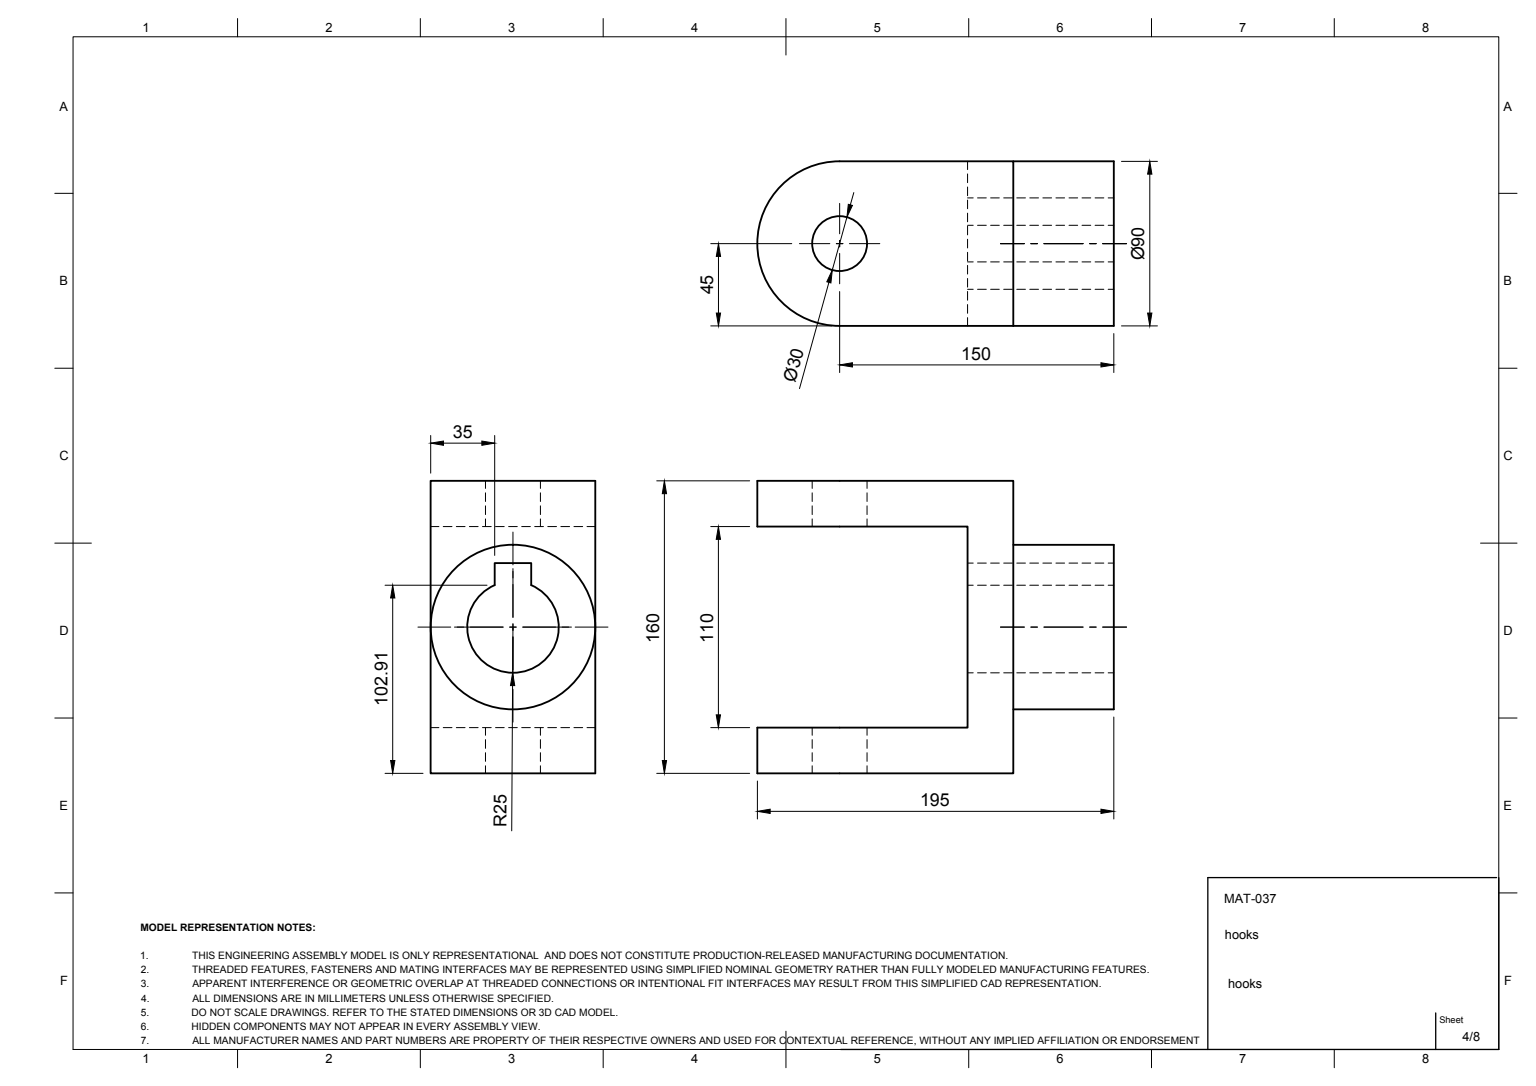
ISO-10303-21;
HEADER;
/* Generated by software containing ST-Developer
 * from STEP Tools, Inc. (www.steptools.com) 
 */

FILE_DESCRIPTION(
/* description */ ('STEP AP214'),
/* implementation_level */ '2;1');

FILE_NAME(
/* name */ 'hooks.step',
/* time_stamp */ '2026-11-14T21:09:07-08:00',
/* author */ (''),
/* organization */ (''),
/* preprocessor_version */ 'ST-DEVELOPER v20.2',
/* originating_system */ 'Autodesk Translation Framework v15.17.0.0',
/* authorisation */ '');

FILE_SCHEMA (('AUTOMOTIVE_DESIGN { 1 0 10303 214 3 1 1 }'));
ENDSEC;

DATA;
#10=MECHANICAL_DESIGN_GEOMETRIC_PRESENTATION_REPRESENTATION('',(#79),#2059);
#65=SHAPE_REPRESENTATION_RELATIONSHIP('SRR','None',#2095,#72);
#72=ADVANCED_BREP_SHAPE_REPRESENTATION('',(#86),#2053);
#79=STYLED_ITEM('',(#2139),#86);
#86=MANIFOLD_SOLID_BREP('Body1',#976);
#96=PLANE('',#1092);
#97=PLANE('',#1093);
#98=PLANE('',#1094);
#99=PLANE('',#1095);
#100=PLANE('',#1097);
#101=PLANE('',#1098);
#102=PLANE('',#1100);
#103=PLANE('',#1102);
#104=PLANE('',#1103);
#105=PLANE('',#1105);
#106=PLANE('',#1108);
#107=PLANE('',#1109);
#108=PLANE('',#1110);
#131=FACE_BOUND('',#234,.T.);
#132=FACE_BOUND('',#237,.T.);
#133=FACE_BOUND('',#239,.T.);
#134=FACE_BOUND('',#241,.T.);
#135=FACE_BOUND('',#243,.T.);
#136=FACE_BOUND('',#245,.T.);
#164=FACE_OUTER_BOUND('',#226,.T.);
#165=FACE_OUTER_BOUND('',#227,.T.);
#166=FACE_OUTER_BOUND('',#228,.T.);
#167=FACE_OUTER_BOUND('',#229,.T.);
#168=FACE_OUTER_BOUND('',#230,.T.);
#169=FACE_OUTER_BOUND('',#231,.T.);
#170=FACE_OUTER_BOUND('',#232,.T.);
#171=FACE_OUTER_BOUND('',#233,.T.);
#172=FACE_OUTER_BOUND('',#235,.T.);
#173=FACE_OUTER_BOUND('',#236,.T.);
#174=FACE_OUTER_BOUND('',#238,.T.);
#175=FACE_OUTER_BOUND('',#240,.T.);
#176=FACE_OUTER_BOUND('',#242,.T.);
#177=FACE_OUTER_BOUND('',#244,.T.);
#178=FACE_OUTER_BOUND('',#246,.T.);
#179=FACE_OUTER_BOUND('',#247,.T.);
#180=FACE_OUTER_BOUND('',#248,.T.);
#181=FACE_OUTER_BOUND('',#249,.T.);
#182=FACE_OUTER_BOUND('',#250,.T.);
#226=EDGE_LOOP('',(#685,#686,#687,#688));
#227=EDGE_LOOP('',(#689,#690,#691,#692));
#228=EDGE_LOOP('',(#693,#694,#695,#696));
#229=EDGE_LOOP('',(#697,#698,#699,#700,#701));
#230=EDGE_LOOP('',(#702,#703,#704,#705,#706,#707,#708,#709,#710));
#231=EDGE_LOOP('',(#711,#712,#713,#714,#715,#716,#717,#718,#719));
#232=EDGE_LOOP('',(#720,#721,#722,#723));
#233=EDGE_LOOP('',(#724,#725,#726,#727));
#234=EDGE_LOOP('',(#728));
#235=EDGE_LOOP('',(#729,#730,#731,#732));
#236=EDGE_LOOP('',(#733,#734,#735,#736));
#237=EDGE_LOOP('',(#737));
#238=EDGE_LOOP('',(#738,#739,#740,#741));
#239=EDGE_LOOP('',(#742));
#240=EDGE_LOOP('',(#743,#744,#745,#746));
#241=EDGE_LOOP('',(#747,#748,#749,#750));
#242=EDGE_LOOP('',(#751,#752,#753,#754));
#243=EDGE_LOOP('',(#755));
#244=EDGE_LOOP('',(#756));
#245=EDGE_LOOP('',(#757,#758,#759,#760));
#246=EDGE_LOOP('',(#761,#762,#763,#764));
#247=EDGE_LOOP('',(#765,#766,#767,#768));
#248=EDGE_LOOP('',(#769,#770,#771,#772));
#249=EDGE_LOOP('',(#773,#774,#775,#776));
#250=EDGE_LOOP('',(#777,#778,#779,#780));
#292=LINE('',#1587,#357);
#293=LINE('',#1593,#358);
#294=LINE('',#1600,#359);
#295=LINE('',#1603,#360);
#296=LINE('',#1609,#361);
#297=LINE('',#1615,#362);
#298=LINE('',#1617,#363);
#299=LINE('',#1619,#364);
#300=LINE('',#1621,#365);
#301=LINE('',#1623,#366);
#302=LINE('',#1625,#367);
#303=LINE('',#1627,#368);
#304=LINE('',#1628,#369);
#305=LINE('',#1629,#370);
#306=LINE('',#1633,#371);
#307=LINE('',#1635,#372);
#308=LINE('',#1636,#373);
#309=LINE('',#1638,#374);
#310=LINE('',#1640,#375);
#311=LINE('',#1642,#376);
#312=LINE('',#1644,#377);
#313=LINE('',#1646,#378);
#314=LINE('',#1647,#379);
#315=LINE('',#1649,#380);
#316=LINE('',#1653,#381);
#317=LINE('',#1658,#382);
#318=LINE('',#1660,#383);
#319=LINE('',#1662,#384);
#320=LINE('',#1664,#385);
#321=LINE('',#1665,#386);
#322=LINE('',#1670,#387);
#323=LINE('',#1672,#388);
#324=LINE('',#1673,#389);
#325=LINE('',#1677,#390);
#326=LINE('',#1679,#391);
#357=VECTOR('',#1226,15.0000000000001);
#358=VECTOR('',#1233,15.0000000000001);
#359=VECTOR('',#1240,1000.);
#360=VECTOR('',#1243,1000.);
#361=VECTOR('',#1248,45.0000000000003);
#362=VECTOR('',#1255,1000.);
#363=VECTOR('',#1256,1000.);
#364=VECTOR('',#1257,1000.);
#365=VECTOR('',#1258,1000.);
#366=VECTOR('',#1259,1000.);
#367=VECTOR('',#1260,1000.);
#368=VECTOR('',#1261,1000.);
#369=VECTOR('',#1262,1000.);
#370=VECTOR('',#1263,1000.);
#371=VECTOR('',#1266,1000.);
#372=VECTOR('',#1267,1000.);
#373=VECTOR('',#1268,1000.);
#374=VECTOR('',#1269,1000.);
#375=VECTOR('',#1270,1000.);
#376=VECTOR('',#1271,1000.);
#377=VECTOR('',#1272,1000.);
#378=VECTOR('',#1273,1000.);
#379=VECTOR('',#1274,1000.);
#380=VECTOR('',#1277,1000.);
#381=VECTOR('',#1284,1000.);
#382=VECTOR('',#1293,1000.);
#383=VECTOR('',#1296,1000.);
#384=VECTOR('',#1297,1000.);
#385=VECTOR('',#1298,1000.);
#386=VECTOR('',#1299,1000.);
#387=VECTOR('',#1306,1000.);
#388=VECTOR('',#1307,1000.);
#389=VECTOR('',#1308,1000.);
#390=VECTOR('',#1315,1000.);
#391=VECTOR('',#1318,1000.);
#426=CIRCLE('',#1080,15.0000000000001);
#427=CIRCLE('',#1081,15.0000000000001);
#428=CIRCLE('',#1083,15.0000000000001);
#429=CIRCLE('',#1084,15.0000000000001);
#430=CIRCLE('',#1086,25.0000000000002);
#431=CIRCLE('',#1087,25.0000000000002);
#432=CIRCLE('',#1089,45.0000000000003);
#433=CIRCLE('',#1090,45.0000000000003);
#434=CIRCLE('',#1091,45.0000000000003);
#435=CIRCLE('',#1096,45.0000000000003);
#436=CIRCLE('',#1099,45.0000000000003);
#437=CIRCLE('',#1101,45.0000000000003);
#438=CIRCLE('',#1104,45.0000000000003);
#470=VERTEX_POINT('',#1584);
#471=VERTEX_POINT('',#1586);
#472=VERTEX_POINT('',#1590);
#473=VERTEX_POINT('',#1592);
#474=VERTEX_POINT('',#1596);
#475=VERTEX_POINT('',#1597);
#476=VERTEX_POINT('',#1599);
#477=VERTEX_POINT('',#1601);
#478=VERTEX_POINT('',#1605);
#479=VERTEX_POINT('',#1606);
#480=VERTEX_POINT('',#1608);
#481=VERTEX_POINT('',#1613);
#482=VERTEX_POINT('',#1614);
#483=VERTEX_POINT('',#1616);
#484=VERTEX_POINT('',#1618);
#485=VERTEX_POINT('',#1620);
#486=VERTEX_POINT('',#1622);
#487=VERTEX_POINT('',#1624);
#488=VERTEX_POINT('',#1626);
#489=VERTEX_POINT('',#1631);
#490=VERTEX_POINT('',#1632);
#491=VERTEX_POINT('',#1634);
#492=VERTEX_POINT('',#1637);
#493=VERTEX_POINT('',#1639);
#494=VERTEX_POINT('',#1641);
#495=VERTEX_POINT('',#1643);
#496=VERTEX_POINT('',#1645);
#497=VERTEX_POINT('',#1661);
#498=VERTEX_POINT('',#1663);
#499=VERTEX_POINT('',#1669);
#500=VERTEX_POINT('',#1671);
#553=EDGE_CURVE('',#470,#470,#426,.T.);
#554=EDGE_CURVE('',#470,#471,#292,.T.);
#555=EDGE_CURVE('',#471,#471,#427,.T.);
#556=EDGE_CURVE('',#472,#472,#428,.T.);
#557=EDGE_CURVE('',#472,#473,#293,.T.);
#558=EDGE_CURVE('',#473,#473,#429,.T.);
#559=EDGE_CURVE('',#474,#475,#430,.T.);
#560=EDGE_CURVE('',#476,#474,#294,.T.);
#561=EDGE_CURVE('',#476,#477,#431,.T.);
#562=EDGE_CURVE('',#475,#477,#295,.T.);
#563=EDGE_CURVE('',#478,#479,#432,.T.);
#564=EDGE_CURVE('',#478,#480,#296,.T.);
#565=EDGE_CURVE('',#480,#480,#433,.T.);
#566=EDGE_CURVE('',#479,#478,#434,.T.);
#567=EDGE_CURVE('',#481,#482,#297,.T.);
#568=EDGE_CURVE('',#482,#483,#298,.T.);
#569=EDGE_CURVE('',#483,#484,#299,.T.);
#570=EDGE_CURVE('',#485,#484,#300,.T.);
#571=EDGE_CURVE('',#485,#486,#301,.T.);
#572=EDGE_CURVE('',#486,#487,#302,.T.);
#573=EDGE_CURVE('',#487,#488,#303,.T.);
#574=EDGE_CURVE('',#488,#478,#304,.T.);
#575=EDGE_CURVE('',#478,#481,#305,.T.);
#576=EDGE_CURVE('',#489,#490,#306,.T.);
#577=EDGE_CURVE('',#491,#489,#307,.T.);
#578=EDGE_CURVE('',#479,#491,#308,.T.);
#579=EDGE_CURVE('',#492,#479,#309,.T.);
#580=EDGE_CURVE('',#493,#492,#310,.T.);
#581=EDGE_CURVE('',#494,#493,#311,.T.);
#582=EDGE_CURVE('',#495,#494,#312,.T.);
#583=EDGE_CURVE('',#495,#496,#313,.T.);
#584=EDGE_CURVE('',#490,#496,#314,.T.);
#585=EDGE_CURVE('',#488,#492,#315,.T.);
#586=EDGE_CURVE('',#493,#487,#435,.T.);
#587=EDGE_CURVE('',#481,#491,#316,.T.);
#588=EDGE_CURVE('',#489,#482,#436,.T.);
#589=EDGE_CURVE('',#483,#490,#437,.T.);
#590=EDGE_CURVE('',#484,#496,#317,.T.);
#591=EDGE_CURVE('',#485,#495,#318,.T.);
#592=EDGE_CURVE('',#477,#497,#319,.T.);
#593=EDGE_CURVE('',#498,#476,#320,.T.);
#594=EDGE_CURVE('',#497,#498,#321,.T.);
#595=EDGE_CURVE('',#494,#486,#438,.T.);
#596=EDGE_CURVE('',#499,#475,#322,.T.);
#597=EDGE_CURVE('',#500,#499,#323,.T.);
#598=EDGE_CURVE('',#474,#500,#324,.T.);
#599=EDGE_CURVE('',#497,#499,#325,.T.);
#600=EDGE_CURVE('',#498,#500,#326,.T.);
#685=ORIENTED_EDGE('',*,*,#553,.F.);
#686=ORIENTED_EDGE('',*,*,#554,.T.);
#687=ORIENTED_EDGE('',*,*,#555,.F.);
#688=ORIENTED_EDGE('',*,*,#554,.F.);
#689=ORIENTED_EDGE('',*,*,#556,.F.);
#690=ORIENTED_EDGE('',*,*,#557,.T.);
#691=ORIENTED_EDGE('',*,*,#558,.T.);
#692=ORIENTED_EDGE('',*,*,#557,.F.);
#693=ORIENTED_EDGE('',*,*,#559,.F.);
#694=ORIENTED_EDGE('',*,*,#560,.F.);
#695=ORIENTED_EDGE('',*,*,#561,.T.);
#696=ORIENTED_EDGE('',*,*,#562,.F.);
#697=ORIENTED_EDGE('',*,*,#563,.F.);
#698=ORIENTED_EDGE('',*,*,#564,.T.);
#699=ORIENTED_EDGE('',*,*,#565,.T.);
#700=ORIENTED_EDGE('',*,*,#564,.F.);
#701=ORIENTED_EDGE('',*,*,#566,.F.);
#702=ORIENTED_EDGE('',*,*,#567,.T.);
#703=ORIENTED_EDGE('',*,*,#568,.T.);
#704=ORIENTED_EDGE('',*,*,#569,.T.);
#705=ORIENTED_EDGE('',*,*,#570,.F.);
#706=ORIENTED_EDGE('',*,*,#571,.T.);
#707=ORIENTED_EDGE('',*,*,#572,.T.);
#708=ORIENTED_EDGE('',*,*,#573,.T.);
#709=ORIENTED_EDGE('',*,*,#574,.T.);
#710=ORIENTED_EDGE('',*,*,#575,.T.);
#711=ORIENTED_EDGE('',*,*,#576,.F.);
#712=ORIENTED_EDGE('',*,*,#577,.F.);
#713=ORIENTED_EDGE('',*,*,#578,.F.);
#714=ORIENTED_EDGE('',*,*,#579,.F.);
#715=ORIENTED_EDGE('',*,*,#580,.F.);
#716=ORIENTED_EDGE('',*,*,#581,.F.);
#717=ORIENTED_EDGE('',*,*,#582,.F.);
#718=ORIENTED_EDGE('',*,*,#583,.T.);
#719=ORIENTED_EDGE('',*,*,#584,.F.);
#720=ORIENTED_EDGE('',*,*,#579,.T.);
#721=ORIENTED_EDGE('',*,*,#566,.T.);
#722=ORIENTED_EDGE('',*,*,#574,.F.);
#723=ORIENTED_EDGE('',*,*,#585,.T.);
#724=ORIENTED_EDGE('',*,*,#573,.F.);
#725=ORIENTED_EDGE('',*,*,#586,.F.);
#726=ORIENTED_EDGE('',*,*,#580,.T.);
#727=ORIENTED_EDGE('',*,*,#585,.F.);
#728=ORIENTED_EDGE('',*,*,#558,.F.);
#729=ORIENTED_EDGE('',*,*,#575,.F.);
#730=ORIENTED_EDGE('',*,*,#563,.T.);
#731=ORIENTED_EDGE('',*,*,#578,.T.);
#732=ORIENTED_EDGE('',*,*,#587,.F.);
#733=ORIENTED_EDGE('',*,*,#577,.T.);
#734=ORIENTED_EDGE('',*,*,#588,.T.);
#735=ORIENTED_EDGE('',*,*,#567,.F.);
#736=ORIENTED_EDGE('',*,*,#587,.T.);
#737=ORIENTED_EDGE('',*,*,#553,.T.);
#738=ORIENTED_EDGE('',*,*,#569,.F.);
#739=ORIENTED_EDGE('',*,*,#589,.T.);
#740=ORIENTED_EDGE('',*,*,#584,.T.);
#741=ORIENTED_EDGE('',*,*,#590,.F.);
#742=ORIENTED_EDGE('',*,*,#555,.T.);
#743=ORIENTED_EDGE('',*,*,#583,.F.);
#744=ORIENTED_EDGE('',*,*,#591,.F.);
#745=ORIENTED_EDGE('',*,*,#570,.T.);
#746=ORIENTED_EDGE('',*,*,#590,.T.);
#747=ORIENTED_EDGE('',*,*,#592,.F.);
#748=ORIENTED_EDGE('',*,*,#561,.F.);
#749=ORIENTED_EDGE('',*,*,#593,.F.);
#750=ORIENTED_EDGE('',*,*,#594,.F.);
#751=ORIENTED_EDGE('',*,*,#582,.T.);
#752=ORIENTED_EDGE('',*,*,#595,.T.);
#753=ORIENTED_EDGE('',*,*,#571,.F.);
#754=ORIENTED_EDGE('',*,*,#591,.T.);
#755=ORIENTED_EDGE('',*,*,#556,.T.);
#756=ORIENTED_EDGE('',*,*,#565,.F.);
#757=ORIENTED_EDGE('',*,*,#596,.F.);
#758=ORIENTED_EDGE('',*,*,#597,.F.);
#759=ORIENTED_EDGE('',*,*,#598,.F.);
#760=ORIENTED_EDGE('',*,*,#559,.T.);
#761=ORIENTED_EDGE('',*,*,#586,.T.);
#762=ORIENTED_EDGE('',*,*,#572,.F.);
#763=ORIENTED_EDGE('',*,*,#595,.F.);
#764=ORIENTED_EDGE('',*,*,#581,.T.);
#765=ORIENTED_EDGE('',*,*,#576,.T.);
#766=ORIENTED_EDGE('',*,*,#589,.F.);
#767=ORIENTED_EDGE('',*,*,#568,.F.);
#768=ORIENTED_EDGE('',*,*,#588,.F.);
#769=ORIENTED_EDGE('',*,*,#592,.T.);
#770=ORIENTED_EDGE('',*,*,#599,.T.);
#771=ORIENTED_EDGE('',*,*,#596,.T.);
#772=ORIENTED_EDGE('',*,*,#562,.T.);
#773=ORIENTED_EDGE('',*,*,#594,.T.);
#774=ORIENTED_EDGE('',*,*,#600,.T.);
#775=ORIENTED_EDGE('',*,*,#597,.T.);
#776=ORIENTED_EDGE('',*,*,#599,.F.);
#777=ORIENTED_EDGE('',*,*,#593,.T.);
#778=ORIENTED_EDGE('',*,*,#560,.T.);
#779=ORIENTED_EDGE('',*,*,#598,.T.);
#780=ORIENTED_EDGE('',*,*,#600,.F.);
#901=CYLINDRICAL_SURFACE('',#1079,15.0000000000001);
#902=CYLINDRICAL_SURFACE('',#1082,15.0000000000001);
#903=CYLINDRICAL_SURFACE('',#1085,25.0000000000002);
#904=CYLINDRICAL_SURFACE('',#1088,45.0000000000003);
#905=CYLINDRICAL_SURFACE('',#1106,45.0000000000003);
#906=CYLINDRICAL_SURFACE('',#1107,45.0000000000003);
#927=ADVANCED_FACE('',(#164),#901,.F.);
#928=ADVANCED_FACE('',(#165),#902,.F.);
#929=ADVANCED_FACE('',(#166),#903,.F.);
#930=ADVANCED_FACE('',(#167),#904,.T.);
#931=ADVANCED_FACE('',(#168),#96,.T.);
#932=ADVANCED_FACE('',(#169),#97,.F.);
#933=ADVANCED_FACE('',(#170),#98,.F.);
#934=ADVANCED_FACE('',(#171,#131),#99,.F.);
#935=ADVANCED_FACE('',(#172),#100,.F.);
#936=ADVANCED_FACE('',(#173,#132),#101,.F.);
#937=ADVANCED_FACE('',(#174,#133),#102,.F.);
#938=ADVANCED_FACE('',(#175,#134),#103,.T.);
#939=ADVANCED_FACE('',(#176,#135),#104,.F.);
#940=ADVANCED_FACE('',(#177,#136),#105,.T.);
#941=ADVANCED_FACE('',(#178),#905,.T.);
#942=ADVANCED_FACE('',(#179),#906,.T.);
#943=ADVANCED_FACE('',(#180),#106,.F.);
#944=ADVANCED_FACE('',(#181),#107,.F.);
#945=ADVANCED_FACE('',(#182),#108,.F.);
#976=CLOSED_SHELL('',(#927,#928,#929,#930,#931,#932,#933,#934,#935,#936,
#937,#938,#939,#940,#941,#942,#943,#944,#945));
#1078=AXIS2_PLACEMENT_3D('',#1582,#1220,#1221);
#1079=AXIS2_PLACEMENT_3D('',#1583,#1222,#1223);
#1080=AXIS2_PLACEMENT_3D('',#1585,#1224,#1225);
#1081=AXIS2_PLACEMENT_3D('',#1588,#1227,#1228);
#1082=AXIS2_PLACEMENT_3D('',#1589,#1229,#1230);
#1083=AXIS2_PLACEMENT_3D('',#1591,#1231,#1232);
#1084=AXIS2_PLACEMENT_3D('',#1594,#1234,#1235);
#1085=AXIS2_PLACEMENT_3D('',#1595,#1236,#1237);
#1086=AXIS2_PLACEMENT_3D('',#1598,#1238,#1239);
#1087=AXIS2_PLACEMENT_3D('',#1602,#1241,#1242);
#1088=AXIS2_PLACEMENT_3D('',#1604,#1244,#1245);
#1089=AXIS2_PLACEMENT_3D('',#1607,#1246,#1247);
#1090=AXIS2_PLACEMENT_3D('',#1610,#1249,#1250);
#1091=AXIS2_PLACEMENT_3D('',#1611,#1251,#1252);
#1092=AXIS2_PLACEMENT_3D('',#1612,#1253,#1254);
#1093=AXIS2_PLACEMENT_3D('',#1630,#1264,#1265);
#1094=AXIS2_PLACEMENT_3D('',#1648,#1275,#1276);
#1095=AXIS2_PLACEMENT_3D('',#1650,#1278,#1279);
#1096=AXIS2_PLACEMENT_3D('',#1651,#1280,#1281);
#1097=AXIS2_PLACEMENT_3D('',#1652,#1282,#1283);
#1098=AXIS2_PLACEMENT_3D('',#1654,#1285,#1286);
#1099=AXIS2_PLACEMENT_3D('',#1655,#1287,#1288);
#1100=AXIS2_PLACEMENT_3D('',#1656,#1289,#1290);
#1101=AXIS2_PLACEMENT_3D('',#1657,#1291,#1292);
#1102=AXIS2_PLACEMENT_3D('',#1659,#1294,#1295);
#1103=AXIS2_PLACEMENT_3D('',#1666,#1300,#1301);
#1104=AXIS2_PLACEMENT_3D('',#1667,#1302,#1303);
#1105=AXIS2_PLACEMENT_3D('',#1668,#1304,#1305);
#1106=AXIS2_PLACEMENT_3D('',#1674,#1309,#1310);
#1107=AXIS2_PLACEMENT_3D('',#1675,#1311,#1312);
#1108=AXIS2_PLACEMENT_3D('',#1676,#1313,#1314);
#1109=AXIS2_PLACEMENT_3D('',#1678,#1316,#1317);
#1110=AXIS2_PLACEMENT_3D('',#1680,#1319,#1320);
#1220=DIRECTION('axis',(0.,0.,1.));
#1221=DIRECTION('refdir',(1.,0.,0.));
#1222=DIRECTION('center_axis',(-8.09275762631517E-30,1.,-3.72243739651165E-30));
#1223=DIRECTION('ref_axis',(-3.01247836291004E-59,3.72243739651165E-30,
1.));
#1224=DIRECTION('center_axis',(-8.09237244032629E-30,1.,-3.72243739651165E-30));
#1225=DIRECTION('ref_axis',(-3.01233497983708E-59,3.72243739651165E-30,
1.));
#1226=DIRECTION('',(-8.09275762631517E-30,1.,-3.72243739651165E-30));
#1227=DIRECTION('center_axis',(8.09237244032629E-30,-1.,3.72243739651165E-30));
#1228=DIRECTION('ref_axis',(3.01233497983708E-59,-3.72243739651165E-30,
-1.));
#1229=DIRECTION('center_axis',(-8.09275762631517E-30,1.,-3.72243739651165E-30));
#1230=DIRECTION('ref_axis',(-3.01247836291004E-59,3.72243739651165E-30,
1.));
#1231=DIRECTION('center_axis',(-8.09237244032629E-30,1.,-3.72243739651165E-30));
#1232=DIRECTION('ref_axis',(-3.01233497983708E-59,3.72243739651165E-30,
1.));
#1233=DIRECTION('',(-8.09275762631517E-30,1.,-3.72243739651165E-30));
#1234=DIRECTION('center_axis',(-8.09275762631517E-30,1.,-3.72243739651165E-30));
#1235=DIRECTION('ref_axis',(-3.01247836291004E-59,3.72243739651165E-30,
1.));
#1236=DIRECTION('center_axis',(1.,-7.90786835165394E-30,1.38777878078144E-17));
#1237=DIRECTION('ref_axis',(-7.96009957174572E-30,-1.,3.7364106986726E-15));
#1238=DIRECTION('center_axis',(1.,-7.90786835165394E-30,1.38777878078144E-17));
#1239=DIRECTION('ref_axis',(1.38777878078144E-17,-1.09743718996384E-46,
-1.));
#1240=DIRECTION('',(-1.,7.90786835165394E-30,-1.38777878078144E-17));
#1241=DIRECTION('center_axis',(1.,-8.05423902742737E-30,1.04083408558608E-17));
#1242=DIRECTION('ref_axis',(1.04083408558608E-17,-8.38312651320406E-47,
-1.));
#1243=DIRECTION('',(1.,-7.90786835165394E-30,1.38777878078144E-17));
#1244=DIRECTION('center_axis',(1.,-7.90786835165394E-30,1.38777878078144E-17));
#1245=DIRECTION('ref_axis',(1.38777878078144E-17,-1.09743718996384E-46,
-1.));
#1246=DIRECTION('center_axis',(1.,-7.90786835165394E-30,1.38777878078144E-17));
#1247=DIRECTION('ref_axis',(1.38777878078144E-17,-1.09743718996384E-46,
-1.));
#1248=DIRECTION('',(-1.,7.90786835165394E-30,-1.38777878078144E-17));
#1249=DIRECTION('center_axis',(1.,-7.90786835165394E-30,1.38777878078144E-17));
#1250=DIRECTION('ref_axis',(1.38777878078144E-17,-1.09743718996384E-46,
-1.));
#1251=DIRECTION('center_axis',(1.,-7.90786835165394E-30,1.38777878078144E-17));
#1252=DIRECTION('ref_axis',(1.38777878078144E-17,-1.09743718996384E-46,
-1.));
#1253=DIRECTION('center_axis',(-1.38777878078144E-17,-3.94430452610503E-30,
1.));
#1254=DIRECTION('ref_axis',(1.,-7.90786835165394E-30,1.38777878078144E-17));
#1255=DIRECTION('',(1.,-7.90786835165394E-30,1.38777878078144E-17));
#1256=DIRECTION('',(-8.09275762631517E-30,1.,-3.72243739651165E-30));
#1257=DIRECTION('',(-1.,7.90786835165394E-30,-1.38777878078144E-17));
#1258=DIRECTION('',(8.09275762631517E-30,-1.,3.72243739651165E-30));
#1259=DIRECTION('',(1.,-7.90786835165394E-30,1.38777878078144E-17));
#1260=DIRECTION('',(-8.09275762631517E-30,1.,-3.72243739651165E-30));
#1261=DIRECTION('',(-1.,7.90786835165394E-30,-1.38777878078144E-17));
#1262=DIRECTION('',(8.09275762631517E-30,-1.,3.72243739651165E-30));
#1263=DIRECTION('',(8.09275762631517E-30,-1.,3.72243739651165E-30));
#1264=DIRECTION('center_axis',(-1.38777878078144E-17,-3.94430452610503E-30,
1.));
#1265=DIRECTION('ref_axis',(1.,-7.90786835165394E-30,1.38777878078144E-17));
#1266=DIRECTION('',(-8.09275762631517E-30,1.,-3.72243739651165E-30));
#1267=DIRECTION('',(1.,-8.05423902742737E-30,1.04083408558608E-17));
#1268=DIRECTION('',(8.09275762631517E-30,-1.,3.72243739651165E-30));
#1269=DIRECTION('',(8.09275762631517E-30,-1.,3.72243739651165E-30));
#1270=DIRECTION('',(-1.,7.90786835165394E-30,-1.38777878078144E-17));
#1271=DIRECTION('',(-8.09275762631517E-30,1.,-3.72243739651165E-30));
#1272=DIRECTION('',(1.,-7.90786835165394E-30,1.38777878078144E-17));
#1273=DIRECTION('',(8.09275762631517E-30,-1.,3.72243739651165E-30));
#1274=DIRECTION('',(-1.,7.90786835165394E-30,-1.38777878078144E-17));
#1275=DIRECTION('center_axis',(1.,-8.05423902742737E-30,1.38777878078144E-17));
#1276=DIRECTION('ref_axis',(1.38777878078144E-17,3.94430452610503E-30,-1.));
#1277=DIRECTION('',(1.04083408558608E-17,3.77174120308794E-30,-1.));
#1278=DIRECTION('center_axis',(8.09237244032629E-30,-1.,-3.94430452610503E-30));
#1279=DIRECTION('ref_axis',(1.38777878078144E-17,3.94430452610503E-30,-1.));
#1280=DIRECTION('center_axis',(8.09275762631517E-30,-1.,3.72243739651165E-30));
#1281=DIRECTION('ref_axis',(-9.8532293435482E-14,3.72243739651085E-30,1.));
#1282=DIRECTION('center_axis',(1.,-8.05423902742737E-30,1.38777878078144E-17));
#1283=DIRECTION('ref_axis',(1.38777878078144E-17,3.94430452610503E-30,-1.));
#1284=DIRECTION('',(1.04083408558608E-17,3.77174120308794E-30,-1.));
#1285=DIRECTION('center_axis',(-8.09237244032629E-30,1.,3.94430452610503E-30));
#1286=DIRECTION('ref_axis',(-1.38777878078144E-17,-3.94430452610503E-30,
1.));
#1287=DIRECTION('center_axis',(8.09237244032629E-30,-1.,3.72243739651165E-30));
#1288=DIRECTION('ref_axis',(-1.87350135405494E-13,3.72243739651013E-30,
1.));
#1289=DIRECTION('center_axis',(8.09237244032629E-30,-1.,-3.94430452610503E-30));
#1290=DIRECTION('ref_axis',(1.38777878078144E-17,3.94430452610503E-30,-1.));
#1291=DIRECTION('center_axis',(-8.09237244032629E-30,1.,-3.72243739651165E-30));
#1292=DIRECTION('ref_axis',(-1.19040579862585E-13,-3.72243739651261E-30,
-1.));
#1293=DIRECTION('',(1.04083408558608E-17,3.77174120308794E-30,-1.));
#1294=DIRECTION('center_axis',(1.,-8.05423902742737E-30,1.38777878078144E-17));
#1295=DIRECTION('ref_axis',(1.38777878078144E-17,3.94430452610503E-30,-1.));
#1296=DIRECTION('',(1.04083408558608E-17,3.77174120308794E-30,-1.));
#1297=DIRECTION('',(-8.09275762631517E-30,1.,-3.72243739651165E-30));
#1298=DIRECTION('',(8.09275762631517E-30,-1.,3.72243739651165E-30));
#1299=DIRECTION('',(-1.38777878078144E-17,-3.94430452610503E-30,1.));
#1300=DIRECTION('center_axis',(-8.09237244032629E-30,1.,3.94430452610503E-30));
#1301=DIRECTION('ref_axis',(-1.38777878078144E-17,-3.94430452610503E-30,
1.));
#1302=DIRECTION('center_axis',(8.09237244032629E-30,-1.,3.72243739651165E-30));
#1303=DIRECTION('ref_axis',(-9.8532293435482E-14,3.72243739651085E-30,1.));
#1304=DIRECTION('center_axis',(-1.,7.90786835165394E-30,-1.38777878078144E-17));
#1305=DIRECTION('ref_axis',(-1.38777878078144E-17,-3.94430452610503E-30,
1.));
#1306=DIRECTION('',(8.09275762631517E-30,-1.,3.72243739651165E-30));
#1307=DIRECTION('',(1.38777878078144E-17,3.94430452610503E-30,-1.));
#1308=DIRECTION('',(-8.09275762631517E-30,1.,-3.72243739651165E-30));
#1309=DIRECTION('center_axis',(-8.09275762631517E-30,1.,-3.72243739651165E-30));
#1310=DIRECTION('ref_axis',(-3.01247836291004E-59,3.72243739651165E-30,
1.));
#1311=DIRECTION('center_axis',(-8.09275762631517E-30,1.,-3.72243739651165E-30));
#1312=DIRECTION('ref_axis',(-3.01247836291004E-59,3.72243739651165E-30,
1.));
#1313=DIRECTION('center_axis',(1.38777878078144E-17,3.94430452610503E-30,
-1.));
#1314=DIRECTION('ref_axis',(-1.,7.90786835165394E-30,-1.38777878078144E-17));
#1315=DIRECTION('',(-1.,7.90786835165394E-30,-1.38777878078144E-17));
#1316=DIRECTION('center_axis',(-8.09275762631516E-30,1.,3.94430452610503E-30));
#1317=DIRECTION('ref_axis',(-1.38777878078144E-17,-3.94430452610503E-30,
1.));
#1318=DIRECTION('',(-1.,7.90786835165394E-30,-1.38777878078144E-17));
#1319=DIRECTION('center_axis',(-1.38777878078144E-17,-3.94430452610503E-30,
1.));
#1320=DIRECTION('ref_axis',(1.,-7.90786835165394E-30,1.38777878078144E-17));
#1582=CARTESIAN_POINT('',(0.,0.,0.));
#1583=CARTESIAN_POINT('Origin',(60.0822225038815,-312.623333755829,0.));
#1584=CARTESIAN_POINT('',(60.0822225038815,-107.623333755829,-15.0000000000001));
#1585=CARTESIAN_POINT('Origin',(60.0822225038811,-107.623333755829,2.22044604925031E-13));
#1586=CARTESIAN_POINT('',(60.0822225038815,-82.6233337558287,-15.0000000000001));
#1587=CARTESIAN_POINT('',(60.0822225038815,-312.623333755829,-15.0000000000001));
#1588=CARTESIAN_POINT('Origin',(60.0822225038811,-82.6233337558288,3.33066907387547E-13));
#1589=CARTESIAN_POINT('Origin',(60.0822225038815,-312.623333755829,0.));
#1590=CARTESIAN_POINT('',(60.0822225038815,27.3766662441712,-15.0000000000001));
#1591=CARTESIAN_POINT('Origin',(60.0822225038811,27.3766662441712,5.55111512312578E-13));
#1592=CARTESIAN_POINT('',(60.0822225038815,52.3766662441712,-15.0000000000001));
#1593=CARTESIAN_POINT('',(60.0822225038815,-312.623333755829,-15.0000000000001));
#1594=CARTESIAN_POINT('Origin',(60.0822225038811,52.3766662441712,4.44089209850063E-13));
#1595=CARTESIAN_POINT('Origin',(-34.9177774961142,-27.6233337558284,-2.22044604925031E-13));
#1596=CARTESIAN_POINT('',(-89.917777496118,-4.71045528104919,9.99999999999956));
#1597=CARTESIAN_POINT('',(-89.9177774961188,-4.71045528104924,-10.0000000000011));
#1598=CARTESIAN_POINT('Origin',(-89.9177774961135,-27.6233337558284,-2.22044604925031E-13));
#1599=CARTESIAN_POINT('',(-9.91777749611433,-4.71045528104919,9.99999999999979));
#1600=CARTESIAN_POINT('',(-34.9177774961102,-4.71045528104919,9.99999999999934));
#1601=CARTESIAN_POINT('',(-9.91777749611433,-4.71045528104919,-10.0000000000002));
#1602=CARTESIAN_POINT('Origin',(-9.91777749611433,-27.6233337558284,7.7715611723761E-13));
#1603=CARTESIAN_POINT('',(-34.9177774961142,-4.71045528104919,-10.));
#1604=CARTESIAN_POINT('Origin',(-34.9177774961142,-27.6233337558284,-2.22044604925031E-13));
#1605=CARTESIAN_POINT('',(-34.9177774961142,-27.6233337558284,44.9999999999998));
#1606=CARTESIAN_POINT('',(-34.9177774961102,-27.6233337558284,-45.0000000000014));
#1607=CARTESIAN_POINT('Origin',(-34.9177774961142,-27.6233337558284,-2.22044604925031E-13));
#1608=CARTESIAN_POINT('',(-89.9177774961135,-27.6233337558284,45.0000000000001));
#1609=CARTESIAN_POINT('',(-34.9177774961142,-27.6233337558284,45.0000000000001));
#1610=CARTESIAN_POINT('Origin',(-89.9177774961135,-27.6233337558284,-2.22044604925031E-13));
#1611=CARTESIAN_POINT('Origin',(-34.9177774961142,-27.6233337558284,-2.22044604925031E-13));
#1612=CARTESIAN_POINT('Origin',(8.88178419700125E-13,0.,44.9999999999998));
#1613=CARTESIAN_POINT('',(-34.9177774961142,-107.623333755829,44.9999999999999));
#1614=CARTESIAN_POINT('',(60.0822225038895,-107.623333755829,44.9999999999998));
#1615=CARTESIAN_POINT('',(-34.9177774961142,-107.623333755829,44.9999999999999));
#1616=CARTESIAN_POINT('',(60.0822225038895,-82.6233337558287,44.9999999999998));
#1617=CARTESIAN_POINT('',(60.08222250389,-312.623333755829,45.0000000000001));
#1618=CARTESIAN_POINT('',(-9.91777749611789,-82.6233337558287,44.9999999999999));
#1619=CARTESIAN_POINT('',(105.082222503891,-82.6233337558287,45.0000000000001));
#1620=CARTESIAN_POINT('',(-9.91777749611789,27.3766662441716,44.9999999999998));
#1621=CARTESIAN_POINT('',(-9.91777749611789,27.3766662441716,44.9999999999998));
#1622=CARTESIAN_POINT('',(60.0822225038855,27.3766662441712,45.));
#1623=CARTESIAN_POINT('',(-9.91777749611789,27.3766662441716,44.9999999999998));
#1624=CARTESIAN_POINT('',(60.0822225038855,52.3766662441712,45.));
#1625=CARTESIAN_POINT('',(60.08222250389,-312.623333755829,45.0000000000001));
#1626=CARTESIAN_POINT('',(-34.9177774961142,52.3766662441716,44.9999999999998));
#1627=CARTESIAN_POINT('',(105.08222250389,52.3766662441715,44.9999999999996));
#1628=CARTESIAN_POINT('',(-34.9177774961142,52.3766662441716,44.9999999999998));
#1629=CARTESIAN_POINT('',(-34.9177774961142,52.3766662441716,44.9999999999998));
#1630=CARTESIAN_POINT('Origin',(-8.43769498715119E-12,0.,-45.0000000000007));
#1631=CARTESIAN_POINT('',(60.0822225038864,-107.623333755829,-45.0000000000001));
#1632=CARTESIAN_POINT('',(60.0822225038864,-82.6233337558288,-45.0000000000001));
#1633=CARTESIAN_POINT('',(60.0822225038864,0.,-45.000000000001));
#1634=CARTESIAN_POINT('',(-34.9177774961102,-107.623333755829,-45.000000000001));
#1635=CARTESIAN_POINT('',(15.0822225038811,-107.623333755829,-45.0000000000004));
#1636=CARTESIAN_POINT('',(-34.9177774961102,-82.623333755829,-45.0000000000012));
#1637=CARTESIAN_POINT('',(-34.9177774961102,52.3766662441717,-45.0000000000012));
#1638=CARTESIAN_POINT('',(-34.9177774961102,-82.623333755829,-45.0000000000012));
#1639=CARTESIAN_POINT('',(60.0822225038864,52.3766662441712,-45.000000000001));
#1640=CARTESIAN_POINT('',(105.082222503885,52.3766662441712,-45.000000000001));
#1641=CARTESIAN_POINT('',(60.0822225038864,27.3766662441712,-45.000000000001));
#1642=CARTESIAN_POINT('',(60.0822225038864,0.,-45.000000000001));
#1643=CARTESIAN_POINT('',(-9.91777749611433,27.3766662441716,-45.0000000000004));
#1644=CARTESIAN_POINT('',(-9.91777749611433,27.3766662441716,-45.0000000000004));
#1645=CARTESIAN_POINT('',(-9.91777749611034,-82.6233337558288,-45.000000000001));
#1646=CARTESIAN_POINT('',(-9.91777749611433,27.3766662441716,-45.0000000000004));
#1647=CARTESIAN_POINT('',(105.082222503886,-82.6233337558288,-45.0000000000004));
#1648=CARTESIAN_POINT('Origin',(-34.9177774961142,-82.6233337558288,44.9999999999998));
#1649=CARTESIAN_POINT('',(-34.9177774961142,52.3766662441716,44.9999999999998));
#1650=CARTESIAN_POINT('Origin',(105.08222250389,52.3766662441715,44.9999999999996));
#1651=CARTESIAN_POINT('Origin',(60.0822225038811,52.3766662441712,4.44089209850063E-13));
#1652=CARTESIAN_POINT('Origin',(-34.9177774961142,-82.6233337558288,44.9999999999998));
#1653=CARTESIAN_POINT('',(-34.9177774961142,-107.623333755829,44.9999999999999));
#1654=CARTESIAN_POINT('Origin',(15.0822225038874,-107.623333755829,45.));
#1655=CARTESIAN_POINT('Origin',(60.0822225038811,-107.623333755829,2.22044604925031E-13));
#1656=CARTESIAN_POINT('Origin',(105.082222503891,-82.6233337558287,45.0000000000001));
#1657=CARTESIAN_POINT('Origin',(60.0822225038811,-82.6233337558288,3.33066907387547E-13));
#1658=CARTESIAN_POINT('',(-9.91777749611789,-82.6233337558287,44.9999999999999));
#1659=CARTESIAN_POINT('Origin',(-9.91777749611789,27.3766662441716,44.9999999999998));
#1660=CARTESIAN_POINT('',(-9.91777749611789,27.3766662441716,44.9999999999998));
#1661=CARTESIAN_POINT('',(-9.91777749611433,7.3766662441716,-10.0000000000002));
#1662=CARTESIAN_POINT('',(-9.91777749611567,27.3766662441716,-10.0000000000002));
#1663=CARTESIAN_POINT('',(-9.91777749611433,7.3766662441716,9.99999999999979));
#1664=CARTESIAN_POINT('',(-9.91777749611433,27.3766662441716,9.99999999999979));
#1665=CARTESIAN_POINT('',(-9.91777749611789,7.3766662441716,44.9999999999998));
#1666=CARTESIAN_POINT('Origin',(-9.91777749611789,27.3766662441716,44.9999999999998));
#1667=CARTESIAN_POINT('Origin',(60.0822225038811,27.3766662441712,5.55111512312578E-13));
#1668=CARTESIAN_POINT('Origin',(-89.917777496114,3.88578058618805E-13,-2.22044604925031E-13));
#1669=CARTESIAN_POINT('',(-89.9177774961188,7.37666624417127,-10.0000000000011));
#1670=CARTESIAN_POINT('',(-89.9177774961188,7.37666624417127,-10.0000000000011));
#1671=CARTESIAN_POINT('',(-89.917777496118,7.3766662441716,9.99999999999956));
#1672=CARTESIAN_POINT('',(-89.9177774961135,7.37666624417133,-2.22044604925031E-13));
#1673=CARTESIAN_POINT('',(-89.917777496118,7.3766662441716,9.99999999999956));
#1674=CARTESIAN_POINT('Origin',(60.0822225038815,-312.623333755829,0.));
#1675=CARTESIAN_POINT('Origin',(60.0822225038815,-312.623333755829,0.));
#1676=CARTESIAN_POINT('Origin',(275.082222503884,7.37666624417121,-10.0000000000003));
#1677=CARTESIAN_POINT('',(275.082222503884,7.37666624417121,-10.0000000000003));
#1678=CARTESIAN_POINT('Origin',(275.082222503886,7.37666624417121,7.7715611723761E-13));
#1679=CARTESIAN_POINT('',(275.082222503887,7.37666624417121,9.9999999999999));
#1680=CARTESIAN_POINT('Origin',(275.082222503887,7.37666624417121,9.9999999999999));
#2044=UNCERTAINTY_MEASURE_WITH_UNIT(LENGTH_MEASURE(0.01),#2060,
'DISTANCE_ACCURACY_VALUE',
'Maximum model space distance between geometric entities at asserted c
onnectivities');
#2050=UNCERTAINTY_MEASURE_WITH_UNIT(LENGTH_MEASURE(0.01),#2060,
'DISTANCE_ACCURACY_VALUE',
'Maximum model space distance between geometric entities at asserted c
onnectivities');
#2053=(
GEOMETRIC_REPRESENTATION_CONTEXT(3)
GLOBAL_UNCERTAINTY_ASSIGNED_CONTEXT((#2044))
GLOBAL_UNIT_ASSIGNED_CONTEXT((#2060,#2062,#2063))
REPRESENTATION_CONTEXT('','3D')
);
#2059=(
GEOMETRIC_REPRESENTATION_CONTEXT(3)
GLOBAL_UNCERTAINTY_ASSIGNED_CONTEXT((#2050))
GLOBAL_UNIT_ASSIGNED_CONTEXT((#2060,#2062,#2063))
REPRESENTATION_CONTEXT('','3D')
);
#2060=(
LENGTH_UNIT()
NAMED_UNIT(*)
SI_UNIT(.MILLI.,.METRE.)
);
#2062=(
NAMED_UNIT(*)
PLANE_ANGLE_UNIT()
SI_UNIT($,.RADIAN.)
);
#2063=(
NAMED_UNIT(*)
SI_UNIT($,.STERADIAN.)
SOLID_ANGLE_UNIT()
);
#2066=SHAPE_DEFINITION_REPRESENTATION(#2074,#2095);
#2074=PRODUCT_DEFINITION_SHAPE('',$,#2104);
#2095=SHAPE_REPRESENTATION('',(#1078),#2053);
#2101=PRODUCT_DEFINITION_CONTEXT('part definition',#2127,'design');
#2104=PRODUCT_DEFINITION('hooks','hooks',#2112,#2101);
#2112=PRODUCT_DEFINITION_FORMATION('',$,#2131);
#2127=APPLICATION_CONTEXT(
'Core Data for Automotive Mechanical Design Process');
#2128=PRODUCT_CONTEXT('part definition',#2127,'mechanical');
#2131=PRODUCT('hooks','hooks',$,(#2128));
#2139=PRESENTATION_STYLE_ASSIGNMENT((#2145));
#2145=SURFACE_STYLE_USAGE(.BOTH.,#2151);
#2151=SURFACE_SIDE_STYLE('',(#2157));
#2157=SURFACE_STYLE_FILL_AREA(#2163);
#2163=FILL_AREA_STYLE('Opaque(61,176,222)',(#2169));
#2169=FILL_AREA_STYLE_COLOUR('Opaque(61,176,222)',#2175);
#2175=COLOUR_RGB('Opaque(61,176,222)',0.23921568627451,0.690196078431373,
0.870588235294118);
ENDSEC;
END-ISO-10303-21;
